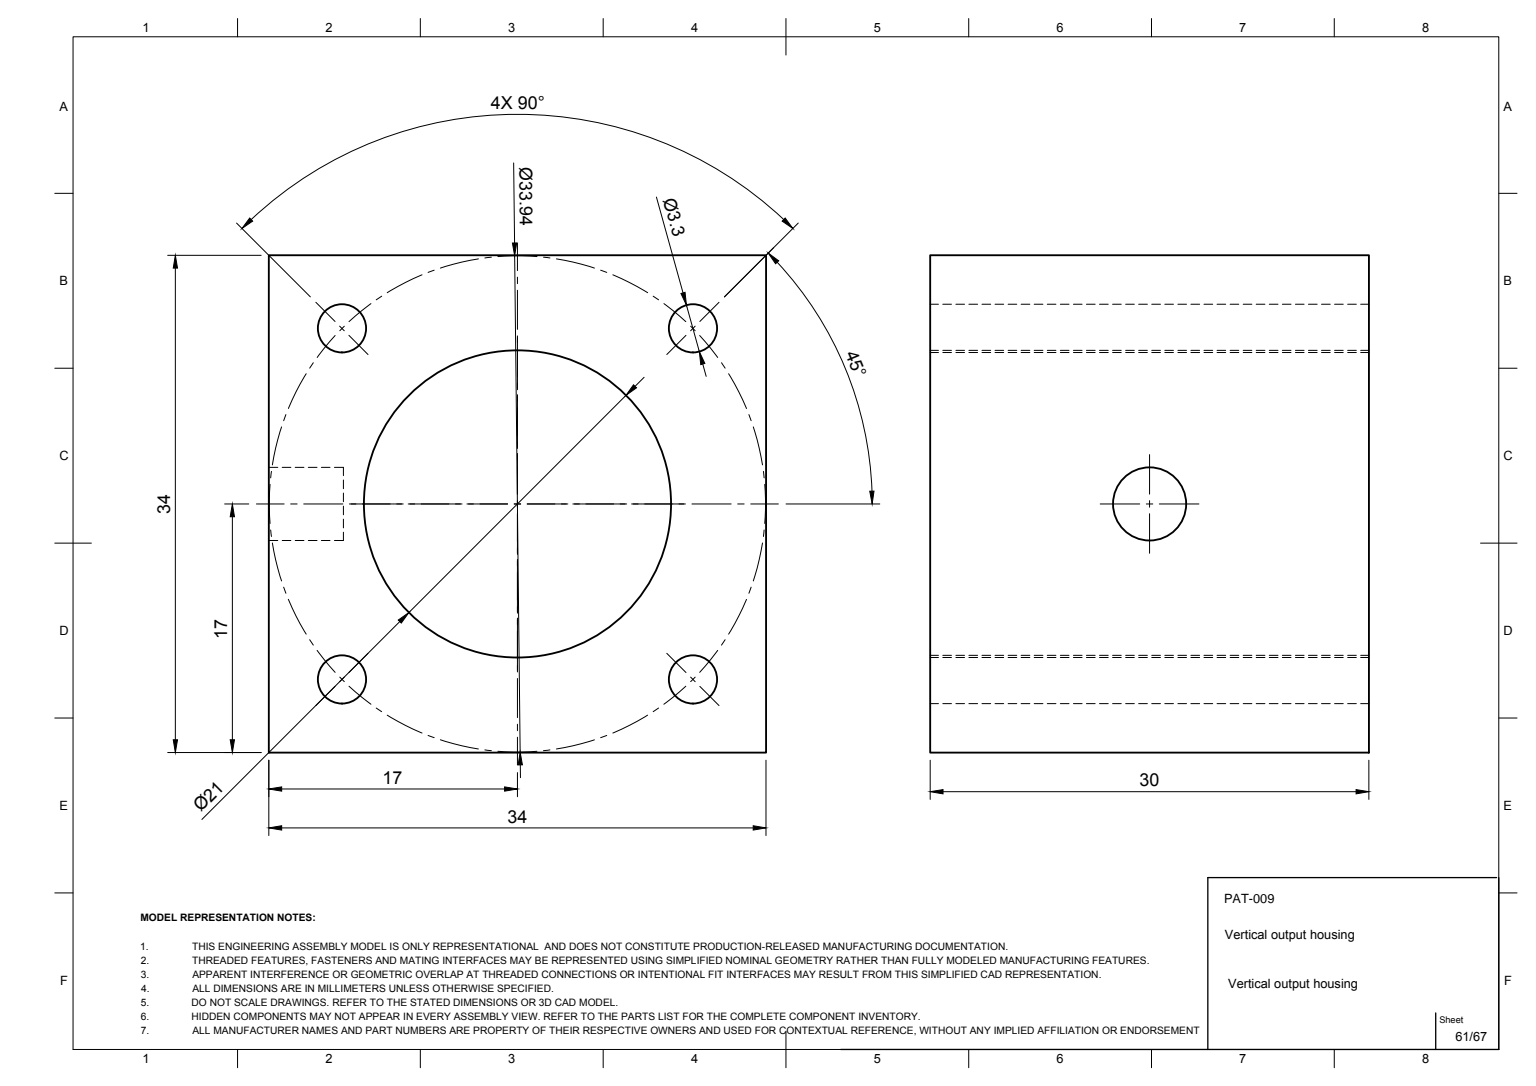
ISO-10303-21;
HEADER;
/* Generated by software containing ST-Developer
 * from STEP Tools, Inc. (www.steptools.com) 
 */

FILE_DESCRIPTION(
/* description */ ('Bell-crank linkage with push rods'),
/* implementation_level */ '2;1');

FILE_NAME(
/* name */ 'Vertical output housing.step',
/* time_stamp */ '2026-10-28T03:25:15-07:00',
/* author */ (''),
/* organization */ (''),
/* preprocessor_version */ 'ST-DEVELOPER v20.2',
/* originating_system */ 'Autodesk Translation Framework v15.17.0.0',
/* authorisation */ '');

FILE_SCHEMA (('AUTOMOTIVE_DESIGN { 1 0 10303 214 3 1 1 }'));
ENDSEC;

DATA;
#10=MECHANICAL_DESIGN_GEOMETRIC_PRESENTATION_REPRESENTATION('',(#656),#16678);
#540=SHAPE_REPRESENTATION_RELATIONSHIP('SRR','None',#16962,#594);
#594=ADVANCED_BREP_SHAPE_REPRESENTATION('',(#716),#16667);
#656=STYLED_ITEM('',(#17270),#716);
#716=MANIFOLD_SOLID_BREP('Body1',#8848);
#914=FACE_BOUND('',#2391,.T.);
#915=FACE_BOUND('',#2392,.T.);
#916=FACE_BOUND('',#2393,.T.);
#917=FACE_BOUND('',#2394,.T.);
#918=FACE_BOUND('',#2395,.T.);
#919=FACE_BOUND('',#2398,.T.);
#920=FACE_BOUND('',#2399,.T.);
#921=FACE_BOUND('',#2400,.T.);
#922=FACE_BOUND('',#2401,.T.);
#923=FACE_BOUND('',#2402,.T.);
#924=FACE_BOUND('',#2405,.T.);
#1189=PLANE('',#10355);
#1190=PLANE('',#10371);
#1191=PLANE('',#10372);
#1192=PLANE('',#10373);
#1193=PLANE('',#10374);
#1194=PLANE('',#10375);
#1195=PLANE('',#10376);
#1672=FACE_OUTER_BOUND('',#2383,.T.);
#1673=FACE_OUTER_BOUND('',#2384,.T.);
#1674=FACE_OUTER_BOUND('',#2385,.T.);
#1675=FACE_OUTER_BOUND('',#2386,.T.);
#1676=FACE_OUTER_BOUND('',#2387,.T.);
#1677=FACE_OUTER_BOUND('',#2388,.T.);
#1678=FACE_OUTER_BOUND('',#2389,.T.);
#1679=FACE_OUTER_BOUND('',#2390,.T.);
#1680=FACE_OUTER_BOUND('',#2396,.T.);
#1681=FACE_OUTER_BOUND('',#2397,.T.);
#1682=FACE_OUTER_BOUND('',#2403,.T.);
#1683=FACE_OUTER_BOUND('',#2404,.T.);
#1684=FACE_OUTER_BOUND('',#2406,.T.);
#2383=EDGE_LOOP('',(#7683,#7684,#7685,#7686));
#2384=EDGE_LOOP('',(#7687));
#2385=EDGE_LOOP('',(#7688,#7689,#7690,#7691));
#2386=EDGE_LOOP('',(#7692,#7693,#7694,#7695));
#2387=EDGE_LOOP('',(#7696,#7697,#7698,#7699));
#2388=EDGE_LOOP('',(#7700,#7701,#7702,#7703));
#2389=EDGE_LOOP('',(#7704,#7705,#7706,#7707));
#2390=EDGE_LOOP('',(#7708,#7709,#7710,#7711));
#2391=EDGE_LOOP('',(#7712));
#2392=EDGE_LOOP('',(#7713));
#2393=EDGE_LOOP('',(#7714));
#2394=EDGE_LOOP('',(#7715));
#2395=EDGE_LOOP('',(#7716));
#2396=EDGE_LOOP('',(#7717,#7718,#7719,#7720));
#2397=EDGE_LOOP('',(#7721,#7722,#7723,#7724));
#2398=EDGE_LOOP('',(#7725));
#2399=EDGE_LOOP('',(#7726));
#2400=EDGE_LOOP('',(#7727));
#2401=EDGE_LOOP('',(#7728));
#2402=EDGE_LOOP('',(#7729));
#2403=EDGE_LOOP('',(#7730,#7731,#7732,#7733));
#2404=EDGE_LOOP('',(#7734,#7735,#7736,#7737));
#2405=EDGE_LOOP('',(#7738));
#2406=EDGE_LOOP('',(#7739,#7740,#7741,#7742));
#2970=LINE('',#16039,#3519);
#2971=LINE('',#16046,#3520);
#2972=LINE('',#16052,#3521);
#2973=LINE('',#16058,#3522);
#2974=LINE('',#16064,#3523);
#2975=LINE('',#16070,#3524);
#2976=LINE('',#16075,#3525);
#2977=LINE('',#16077,#3526);
#2978=LINE('',#16079,#3527);
#2979=LINE('',#16080,#3528);
#2980=LINE('',#16083,#3529);
#2981=LINE('',#16085,#3530);
#2982=LINE('',#16086,#3531);
#2983=LINE('',#16089,#3532);
#2984=LINE('',#16091,#3533);
#2985=LINE('',#16092,#3534);
#2986=LINE('',#16094,#3535);
#2987=LINE('',#16095,#3536);
#3519=VECTOR('',#12868,0.25);
#3520=VECTOR('',#12877,0.165);
#3521=VECTOR('',#12884,0.165);
#3522=VECTOR('',#12891,0.165);
#3523=VECTOR('',#12898,0.165);
#3524=VECTOR('',#12905,1.05);
#3525=VECTOR('',#12910,1.);
#3526=VECTOR('',#12911,1.);
#3527=VECTOR('',#12912,1.);
#3528=VECTOR('',#12913,1.);
#3529=VECTOR('',#12916,1.);
#3530=VECTOR('',#12917,1.);
#3531=VECTOR('',#12918,1.);
#3532=VECTOR('',#12921,1.);
#3533=VECTOR('',#12922,1.);
#3534=VECTOR('',#12923,1.);
#3535=VECTOR('',#12926,1.);
#3536=VECTOR('',#12927,1.);
#4039=CIRCLE('',#10353,0.25);
#4040=CIRCLE('',#10354,0.25);
#4041=CIRCLE('',#10357,0.165);
#4042=CIRCLE('',#10358,0.165);
#4043=CIRCLE('',#10360,0.165);
#4044=CIRCLE('',#10361,0.165);
#4045=CIRCLE('',#10363,0.165);
#4046=CIRCLE('',#10364,0.165);
#4047=CIRCLE('',#10366,0.165);
#4048=CIRCLE('',#10367,0.165);
#4049=CIRCLE('',#10369,1.05);
#4050=CIRCLE('',#10370,1.05);
#4706=VERTEX_POINT('',#16036);
#4707=VERTEX_POINT('',#16038);
#4708=VERTEX_POINT('',#16043);
#4709=VERTEX_POINT('',#16045);
#4710=VERTEX_POINT('',#16049);
#4711=VERTEX_POINT('',#16051);
#4712=VERTEX_POINT('',#16055);
#4713=VERTEX_POINT('',#16057);
#4714=VERTEX_POINT('',#16061);
#4715=VERTEX_POINT('',#16063);
#4716=VERTEX_POINT('',#16067);
#4717=VERTEX_POINT('',#16069);
#4718=VERTEX_POINT('',#16073);
#4719=VERTEX_POINT('',#16074);
#4720=VERTEX_POINT('',#16076);
#4721=VERTEX_POINT('',#16078);
#4722=VERTEX_POINT('',#16082);
#4723=VERTEX_POINT('',#16084);
#4724=VERTEX_POINT('',#16088);
#4725=VERTEX_POINT('',#16090);
#5719=EDGE_CURVE('',#4706,#4706,#4039,.T.);
#5720=EDGE_CURVE('',#4706,#4707,#2970,.T.);
#5721=EDGE_CURVE('',#4707,#4707,#4040,.T.);
#5722=EDGE_CURVE('',#4708,#4708,#4041,.T.);
#5723=EDGE_CURVE('',#4708,#4709,#2971,.T.);
#5724=EDGE_CURVE('',#4709,#4709,#4042,.T.);
#5725=EDGE_CURVE('',#4710,#4710,#4043,.T.);
#5726=EDGE_CURVE('',#4710,#4711,#2972,.T.);
#5727=EDGE_CURVE('',#4711,#4711,#4044,.T.);
#5728=EDGE_CURVE('',#4712,#4712,#4045,.T.);
#5729=EDGE_CURVE('',#4712,#4713,#2973,.T.);
#5730=EDGE_CURVE('',#4713,#4713,#4046,.T.);
#5731=EDGE_CURVE('',#4714,#4714,#4047,.T.);
#5732=EDGE_CURVE('',#4714,#4715,#2974,.T.);
#5733=EDGE_CURVE('',#4715,#4715,#4048,.T.);
#5734=EDGE_CURVE('',#4716,#4716,#4049,.T.);
#5735=EDGE_CURVE('',#4716,#4717,#2975,.T.);
#5736=EDGE_CURVE('',#4717,#4717,#4050,.T.);
#5737=EDGE_CURVE('',#4718,#4719,#2976,.T.);
#5738=EDGE_CURVE('',#4719,#4720,#2977,.T.);
#5739=EDGE_CURVE('',#4721,#4720,#2978,.T.);
#5740=EDGE_CURVE('',#4718,#4721,#2979,.T.);
#5741=EDGE_CURVE('',#4722,#4718,#2980,.T.);
#5742=EDGE_CURVE('',#4723,#4721,#2981,.T.);
#5743=EDGE_CURVE('',#4722,#4723,#2982,.T.);
#5744=EDGE_CURVE('',#4724,#4722,#2983,.T.);
#5745=EDGE_CURVE('',#4725,#4723,#2984,.T.);
#5746=EDGE_CURVE('',#4724,#4725,#2985,.T.);
#5747=EDGE_CURVE('',#4719,#4724,#2986,.T.);
#5748=EDGE_CURVE('',#4720,#4725,#2987,.T.);
#7683=ORIENTED_EDGE('',*,*,#5719,.F.);
#7684=ORIENTED_EDGE('',*,*,#5720,.T.);
#7685=ORIENTED_EDGE('',*,*,#5721,.F.);
#7686=ORIENTED_EDGE('',*,*,#5720,.F.);
#7687=ORIENTED_EDGE('',*,*,#5719,.T.);
#7688=ORIENTED_EDGE('',*,*,#5722,.F.);
#7689=ORIENTED_EDGE('',*,*,#5723,.T.);
#7690=ORIENTED_EDGE('',*,*,#5724,.F.);
#7691=ORIENTED_EDGE('',*,*,#5723,.F.);
#7692=ORIENTED_EDGE('',*,*,#5725,.F.);
#7693=ORIENTED_EDGE('',*,*,#5726,.T.);
#7694=ORIENTED_EDGE('',*,*,#5727,.F.);
#7695=ORIENTED_EDGE('',*,*,#5726,.F.);
#7696=ORIENTED_EDGE('',*,*,#5728,.F.);
#7697=ORIENTED_EDGE('',*,*,#5729,.T.);
#7698=ORIENTED_EDGE('',*,*,#5730,.F.);
#7699=ORIENTED_EDGE('',*,*,#5729,.F.);
#7700=ORIENTED_EDGE('',*,*,#5731,.F.);
#7701=ORIENTED_EDGE('',*,*,#5732,.T.);
#7702=ORIENTED_EDGE('',*,*,#5733,.F.);
#7703=ORIENTED_EDGE('',*,*,#5732,.F.);
#7704=ORIENTED_EDGE('',*,*,#5734,.F.);
#7705=ORIENTED_EDGE('',*,*,#5735,.T.);
#7706=ORIENTED_EDGE('',*,*,#5736,.F.);
#7707=ORIENTED_EDGE('',*,*,#5735,.F.);
#7708=ORIENTED_EDGE('',*,*,#5737,.T.);
#7709=ORIENTED_EDGE('',*,*,#5738,.T.);
#7710=ORIENTED_EDGE('',*,*,#5739,.F.);
#7711=ORIENTED_EDGE('',*,*,#5740,.F.);
#7712=ORIENTED_EDGE('',*,*,#5736,.T.);
#7713=ORIENTED_EDGE('',*,*,#5733,.T.);
#7714=ORIENTED_EDGE('',*,*,#5730,.T.);
#7715=ORIENTED_EDGE('',*,*,#5727,.T.);
#7716=ORIENTED_EDGE('',*,*,#5724,.T.);
#7717=ORIENTED_EDGE('',*,*,#5741,.T.);
#7718=ORIENTED_EDGE('',*,*,#5740,.T.);
#7719=ORIENTED_EDGE('',*,*,#5742,.F.);
#7720=ORIENTED_EDGE('',*,*,#5743,.F.);
#7721=ORIENTED_EDGE('',*,*,#5744,.T.);
#7722=ORIENTED_EDGE('',*,*,#5743,.T.);
#7723=ORIENTED_EDGE('',*,*,#5745,.F.);
#7724=ORIENTED_EDGE('',*,*,#5746,.F.);
#7725=ORIENTED_EDGE('',*,*,#5734,.T.);
#7726=ORIENTED_EDGE('',*,*,#5731,.T.);
#7727=ORIENTED_EDGE('',*,*,#5728,.T.);
#7728=ORIENTED_EDGE('',*,*,#5725,.T.);
#7729=ORIENTED_EDGE('',*,*,#5722,.T.);
#7730=ORIENTED_EDGE('',*,*,#5747,.T.);
#7731=ORIENTED_EDGE('',*,*,#5746,.T.);
#7732=ORIENTED_EDGE('',*,*,#5748,.F.);
#7733=ORIENTED_EDGE('',*,*,#5738,.F.);
#7734=ORIENTED_EDGE('',*,*,#5748,.T.);
#7735=ORIENTED_EDGE('',*,*,#5745,.T.);
#7736=ORIENTED_EDGE('',*,*,#5742,.T.);
#7737=ORIENTED_EDGE('',*,*,#5739,.T.);
#7738=ORIENTED_EDGE('',*,*,#5721,.T.);
#7739=ORIENTED_EDGE('',*,*,#5747,.F.);
#7740=ORIENTED_EDGE('',*,*,#5737,.F.);
#7741=ORIENTED_EDGE('',*,*,#5741,.F.);
#7742=ORIENTED_EDGE('',*,*,#5744,.F.);
#8236=CYLINDRICAL_SURFACE('',#10352,0.25);
#8237=CYLINDRICAL_SURFACE('',#10356,0.165);
#8238=CYLINDRICAL_SURFACE('',#10359,0.165);
#8239=CYLINDRICAL_SURFACE('',#10362,0.165);
#8240=CYLINDRICAL_SURFACE('',#10365,0.165);
#8241=CYLINDRICAL_SURFACE('',#10368,1.05);
#8697=ADVANCED_FACE('',(#1672),#8236,.F.);
#8698=ADVANCED_FACE('',(#1673),#1189,.T.);
#8699=ADVANCED_FACE('',(#1674),#8237,.F.);
#8700=ADVANCED_FACE('',(#1675),#8238,.F.);
#8701=ADVANCED_FACE('',(#1676),#8239,.F.);
#8702=ADVANCED_FACE('',(#1677),#8240,.F.);
#8703=ADVANCED_FACE('',(#1678),#8241,.F.);
#8704=ADVANCED_FACE('',(#1679,#914,#915,#916,#917,#918),#1190,.T.);
#8705=ADVANCED_FACE('',(#1680),#1191,.T.);
#8706=ADVANCED_FACE('',(#1681,#919,#920,#921,#922,#923),#1192,.T.);
#8707=ADVANCED_FACE('',(#1682),#1193,.T.);
#8708=ADVANCED_FACE('',(#1683,#924),#1194,.T.);
#8709=ADVANCED_FACE('',(#1684),#1195,.F.);
#8848=CLOSED_SHELL('',(#8697,#8698,#8699,#8700,#8701,#8702,#8703,#8704,
#8705,#8706,#8707,#8708,#8709));
#10351=AXIS2_PLACEMENT_3D('',#16034,#12862,#12863);
#10352=AXIS2_PLACEMENT_3D('',#16035,#12864,#12865);
#10353=AXIS2_PLACEMENT_3D('',#16037,#12866,#12867);
#10354=AXIS2_PLACEMENT_3D('',#16040,#12869,#12870);
#10355=AXIS2_PLACEMENT_3D('',#16041,#12871,#12872);
#10356=AXIS2_PLACEMENT_3D('',#16042,#12873,#12874);
#10357=AXIS2_PLACEMENT_3D('',#16044,#12875,#12876);
#10358=AXIS2_PLACEMENT_3D('',#16047,#12878,#12879);
#10359=AXIS2_PLACEMENT_3D('',#16048,#12880,#12881);
#10360=AXIS2_PLACEMENT_3D('',#16050,#12882,#12883);
#10361=AXIS2_PLACEMENT_3D('',#16053,#12885,#12886);
#10362=AXIS2_PLACEMENT_3D('',#16054,#12887,#12888);
#10363=AXIS2_PLACEMENT_3D('',#16056,#12889,#12890);
#10364=AXIS2_PLACEMENT_3D('',#16059,#12892,#12893);
#10365=AXIS2_PLACEMENT_3D('',#16060,#12894,#12895);
#10366=AXIS2_PLACEMENT_3D('',#16062,#12896,#12897);
#10367=AXIS2_PLACEMENT_3D('',#16065,#12899,#12900);
#10368=AXIS2_PLACEMENT_3D('',#16066,#12901,#12902);
#10369=AXIS2_PLACEMENT_3D('',#16068,#12903,#12904);
#10370=AXIS2_PLACEMENT_3D('',#16071,#12906,#12907);
#10371=AXIS2_PLACEMENT_3D('',#16072,#12908,#12909);
#10372=AXIS2_PLACEMENT_3D('',#16081,#12914,#12915);
#10373=AXIS2_PLACEMENT_3D('',#16087,#12919,#12920);
#10374=AXIS2_PLACEMENT_3D('',#16093,#12924,#12925);
#10375=AXIS2_PLACEMENT_3D('',#16096,#12928,#12929);
#10376=AXIS2_PLACEMENT_3D('',#16097,#12930,#12931);
#12862=DIRECTION('axis',(0.,0.,1.));
#12863=DIRECTION('refdir',(1.,0.,0.));
#12864=DIRECTION('center_axis',(0.,0.,1.));
#12865=DIRECTION('ref_axis',(1.,0.,0.));
#12866=DIRECTION('center_axis',(0.,0.,1.));
#12867=DIRECTION('ref_axis',(1.,0.,0.));
#12868=DIRECTION('',(0.,0.,1.));
#12869=DIRECTION('center_axis',(0.,0.,-1.));
#12870=DIRECTION('ref_axis',(1.,0.,0.));
#12871=DIRECTION('center_axis',(0.,0.,1.));
#12872=DIRECTION('ref_axis',(1.,0.,0.));
#12873=DIRECTION('center_axis',(0.,1.,0.));
#12874=DIRECTION('ref_axis',(1.,0.,0.));
#12875=DIRECTION('center_axis',(0.,1.,0.));
#12876=DIRECTION('ref_axis',(1.,0.,0.));
#12877=DIRECTION('',(0.,1.,0.));
#12878=DIRECTION('center_axis',(0.,-1.,0.));
#12879=DIRECTION('ref_axis',(1.,0.,0.));
#12880=DIRECTION('center_axis',(0.,1.,0.));
#12881=DIRECTION('ref_axis',(1.,0.,0.));
#12882=DIRECTION('center_axis',(0.,1.,0.));
#12883=DIRECTION('ref_axis',(1.,0.,0.));
#12884=DIRECTION('',(0.,1.,0.));
#12885=DIRECTION('center_axis',(0.,-1.,0.));
#12886=DIRECTION('ref_axis',(1.,0.,0.));
#12887=DIRECTION('center_axis',(0.,1.,0.));
#12888=DIRECTION('ref_axis',(1.,0.,0.));
#12889=DIRECTION('center_axis',(0.,1.,0.));
#12890=DIRECTION('ref_axis',(1.,0.,0.));
#12891=DIRECTION('',(0.,1.,0.));
#12892=DIRECTION('center_axis',(0.,-1.,0.));
#12893=DIRECTION('ref_axis',(1.,0.,0.));
#12894=DIRECTION('center_axis',(0.,1.,0.));
#12895=DIRECTION('ref_axis',(1.,0.,0.));
#12896=DIRECTION('center_axis',(0.,1.,0.));
#12897=DIRECTION('ref_axis',(1.,0.,0.));
#12898=DIRECTION('',(0.,1.,0.));
#12899=DIRECTION('center_axis',(0.,-1.,0.));
#12900=DIRECTION('ref_axis',(1.,0.,0.));
#12901=DIRECTION('center_axis',(0.,1.,0.));
#12902=DIRECTION('ref_axis',(1.,0.,0.));
#12903=DIRECTION('center_axis',(0.,1.,0.));
#12904=DIRECTION('ref_axis',(1.,0.,0.));
#12905=DIRECTION('',(0.,1.,0.));
#12906=DIRECTION('center_axis',(0.,-1.,0.));
#12907=DIRECTION('ref_axis',(1.,0.,0.));
#12908=DIRECTION('center_axis',(0.,1.,0.));
#12909=DIRECTION('ref_axis',(-1.,0.,0.));
#12910=DIRECTION('',(-1.,0.,0.));
#12911=DIRECTION('',(0.,0.,1.));
#12912=DIRECTION('',(-1.,0.,0.));
#12913=DIRECTION('',(0.,0.,1.));
#12914=DIRECTION('center_axis',(1.,0.,0.));
#12915=DIRECTION('ref_axis',(0.,1.,0.));
#12916=DIRECTION('',(0.,1.,0.));
#12917=DIRECTION('',(0.,1.,0.));
#12918=DIRECTION('',(0.,0.,1.));
#12919=DIRECTION('center_axis',(0.,-1.,0.));
#12920=DIRECTION('ref_axis',(1.,0.,0.));
#12921=DIRECTION('',(1.,0.,0.));
#12922=DIRECTION('',(1.,0.,0.));
#12923=DIRECTION('',(0.,0.,1.));
#12924=DIRECTION('center_axis',(-1.,0.,0.));
#12925=DIRECTION('ref_axis',(0.,-1.,0.));
#12926=DIRECTION('',(0.,-1.,0.));
#12927=DIRECTION('',(0.,-1.,0.));
#12928=DIRECTION('center_axis',(0.,0.,1.));
#12929=DIRECTION('ref_axis',(1.,0.,0.));
#12930=DIRECTION('center_axis',(0.,0.,1.));
#12931=DIRECTION('ref_axis',(1.,0.,0.));
#16034=CARTESIAN_POINT('',(0.,0.,0.));
#16035=CARTESIAN_POINT('Origin',(4.,12.,5.19));
#16036=CARTESIAN_POINT('',(3.75,12.,5.19));
#16037=CARTESIAN_POINT('Origin',(4.,12.,5.19));
#16038=CARTESIAN_POINT('',(3.75,12.,5.7));
#16039=CARTESIAN_POINT('',(3.75,12.,5.19));
#16040=CARTESIAN_POINT('Origin',(4.,12.,5.7));
#16041=CARTESIAN_POINT('Origin',(4.,12.,5.19));
#16042=CARTESIAN_POINT('Origin',(5.2,10.4,2.8));
#16043=CARTESIAN_POINT('',(5.035,10.5,2.8));
#16044=CARTESIAN_POINT('Origin',(5.2,10.5,2.8));
#16045=CARTESIAN_POINT('',(5.035,13.5,2.8));
#16046=CARTESIAN_POINT('',(5.035,10.4,2.8));
#16047=CARTESIAN_POINT('Origin',(5.2,13.5,2.8));
#16048=CARTESIAN_POINT('Origin',(2.8,10.4,5.2));
#16049=CARTESIAN_POINT('',(2.635,10.5,5.2));
#16050=CARTESIAN_POINT('Origin',(2.8,10.5,5.2));
#16051=CARTESIAN_POINT('',(2.635,13.5,5.2));
#16052=CARTESIAN_POINT('',(2.635,10.4,5.2));
#16053=CARTESIAN_POINT('Origin',(2.8,13.5,5.2));
#16054=CARTESIAN_POINT('Origin',(2.8,10.4,2.8));
#16055=CARTESIAN_POINT('',(2.635,10.5,2.8));
#16056=CARTESIAN_POINT('Origin',(2.8,10.5,2.8));
#16057=CARTESIAN_POINT('',(2.635,13.5,2.8));
#16058=CARTESIAN_POINT('',(2.635,10.4,2.8));
#16059=CARTESIAN_POINT('Origin',(2.8,13.5,2.8));
#16060=CARTESIAN_POINT('Origin',(5.2,10.4,5.2));
#16061=CARTESIAN_POINT('',(5.035,10.5,5.2));
#16062=CARTESIAN_POINT('Origin',(5.2,10.5,5.2));
#16063=CARTESIAN_POINT('',(5.035,13.5,5.2));
#16064=CARTESIAN_POINT('',(5.035,10.4,5.2));
#16065=CARTESIAN_POINT('Origin',(5.2,13.5,5.2));
#16066=CARTESIAN_POINT('Origin',(4.,10.4,4.));
#16067=CARTESIAN_POINT('',(2.95,10.5,4.));
#16068=CARTESIAN_POINT('Origin',(4.,10.5,4.));
#16069=CARTESIAN_POINT('',(2.95,13.5,4.));
#16070=CARTESIAN_POINT('',(2.95,10.4,4.));
#16071=CARTESIAN_POINT('Origin',(4.,13.5,4.));
#16072=CARTESIAN_POINT('Origin',(5.7,13.5,2.3));
#16073=CARTESIAN_POINT('',(5.7,13.5,2.3));
#16074=CARTESIAN_POINT('',(2.3,13.5,2.3));
#16075=CARTESIAN_POINT('',(5.7,13.5,2.3));
#16076=CARTESIAN_POINT('',(2.3,13.5,5.7));
#16077=CARTESIAN_POINT('',(2.3,13.5,2.3));
#16078=CARTESIAN_POINT('',(5.7,13.5,5.7));
#16079=CARTESIAN_POINT('',(5.7,13.5,5.7));
#16080=CARTESIAN_POINT('',(5.7,13.5,2.3));
#16081=CARTESIAN_POINT('Origin',(5.7,10.5,2.3));
#16082=CARTESIAN_POINT('',(5.7,10.5,2.3));
#16083=CARTESIAN_POINT('',(5.7,10.5,2.3));
#16084=CARTESIAN_POINT('',(5.7,10.5,5.7));
#16085=CARTESIAN_POINT('',(5.7,10.5,5.7));
#16086=CARTESIAN_POINT('',(5.7,10.5,2.3));
#16087=CARTESIAN_POINT('Origin',(2.3,10.5,2.3));
#16088=CARTESIAN_POINT('',(2.3,10.5,2.3));
#16089=CARTESIAN_POINT('',(2.3,10.5,2.3));
#16090=CARTESIAN_POINT('',(2.3,10.5,5.7));
#16091=CARTESIAN_POINT('',(2.3,10.5,5.7));
#16092=CARTESIAN_POINT('',(2.3,10.5,2.3));
#16093=CARTESIAN_POINT('Origin',(2.3,13.5,2.3));
#16094=CARTESIAN_POINT('',(2.3,13.5,2.3));
#16095=CARTESIAN_POINT('',(2.3,13.5,5.7));
#16096=CARTESIAN_POINT('Origin',(4.,12.,5.7));
#16097=CARTESIAN_POINT('Origin',(4.,12.,2.3));
#16603=UNCERTAINTY_MEASURE_WITH_UNIT(LENGTH_MEASURE(0.001),#16679,
'DISTANCE_ACCURACY_VALUE',
'Maximum model space distance between geometric entities at asserted c
onnectivities');
#16614=UNCERTAINTY_MEASURE_WITH_UNIT(LENGTH_MEASURE(0.001),#16679,
'DISTANCE_ACCURACY_VALUE',
'Maximum model space distance between geometric entities at asserted c
onnectivities');
#16667=(
GEOMETRIC_REPRESENTATION_CONTEXT(3)
GLOBAL_UNCERTAINTY_ASSIGNED_CONTEXT((#16603))
GLOBAL_UNIT_ASSIGNED_CONTEXT((#16679,#16681,#16682))
REPRESENTATION_CONTEXT('','3D')
);
#16678=(
GEOMETRIC_REPRESENTATION_CONTEXT(3)
GLOBAL_UNCERTAINTY_ASSIGNED_CONTEXT((#16614))
GLOBAL_UNIT_ASSIGNED_CONTEXT((#16679,#16681,#16682))
REPRESENTATION_CONTEXT('','3D')
);
#16679=(
LENGTH_UNIT()
NAMED_UNIT(*)
SI_UNIT(.CENTI.,.METRE.)
);
#16681=(
NAMED_UNIT(*)
PLANE_ANGLE_UNIT()
SI_UNIT($,.RADIAN.)
);
#16682=(
NAMED_UNIT(*)
SI_UNIT($,.STERADIAN.)
SOLID_ANGLE_UNIT()
);
#16735=SHAPE_DEFINITION_REPRESENTATION(#16809,#16962);
#16809=PRODUCT_DEFINITION_SHAPE('',$,#17026);
#16962=SHAPE_REPRESENTATION('',(#10351),#16667);
#16973=PRODUCT_DEFINITION_CONTEXT('part definition',#17164,'design');
#17026=PRODUCT_DEFINITION('Vertical output housing',
'Vertical output housing',#17089,#16973);
#17089=PRODUCT_DEFINITION_FORMATION('',$,#17218);
#17164=APPLICATION_CONTEXT(
'Core Data for Automotive Mechanical Design Process');
#17165=PRODUCT_CONTEXT('part definition',#17164,'mechanical');
#17218=PRODUCT('Vertical output housing','Vertical output housing',
'Vertical output housing',(#17165));
#17264=COLOUR_RGB('Dark Blue',0.08,0.2,0.34);
#17265=FILL_AREA_STYLE_COLOUR('',#17264);
#17266=FILL_AREA_STYLE('',(#17265));
#17267=SURFACE_STYLE_FILL_AREA(#17266);
#17268=SURFACE_SIDE_STYLE('',(#17267));
#17269=SURFACE_STYLE_USAGE(.BOTH.,#17268);
#17270=PRESENTATION_STYLE_ASSIGNMENT((#17269));
ENDSEC;
END-ISO-10303-21;
